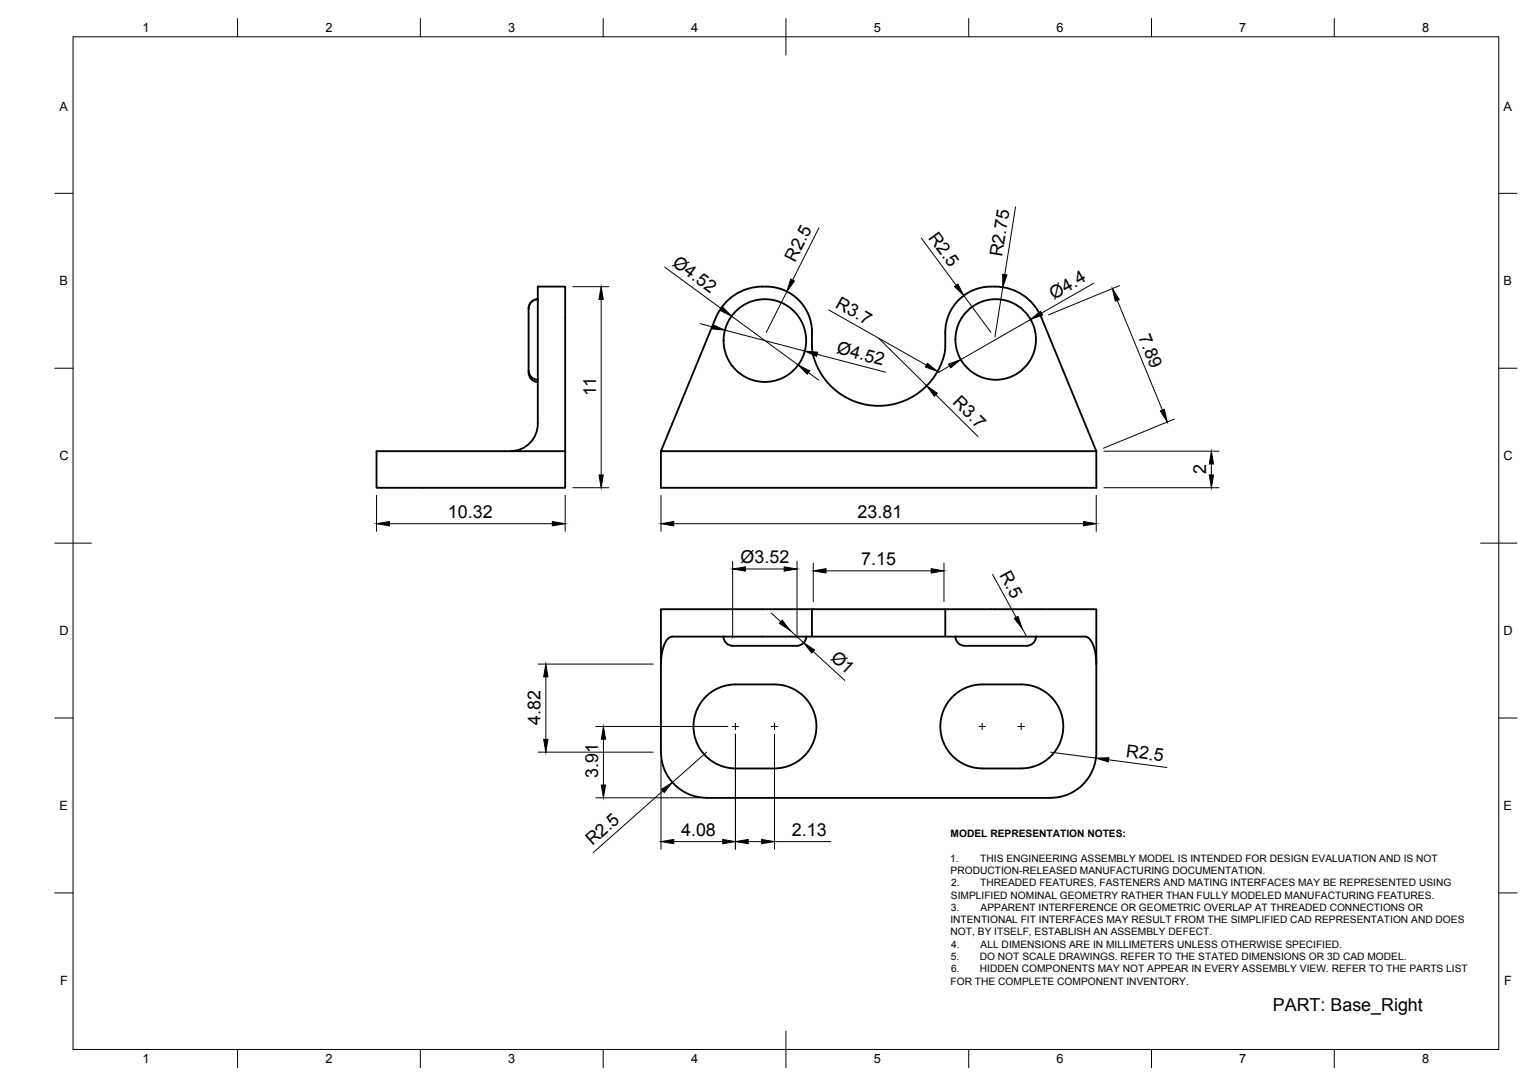
ISO-10303-21;
HEADER;
/* Generated by software containing ST-Developer
 * from STEP Tools, Inc. (www.steptools.com) 
 */

FILE_DESCRIPTION(
/* description */ (''),
/* implementation_level */ '2;1');

FILE_NAME(
/* name */ 'Base_Right.step',
/* time_stamp */ '2026-10-05T16:20:14-07:00',
/* author */ (''),
/* organization */ (''),
/* preprocessor_version */ 'ST-DEVELOPER v20.2',
/* originating_system */ 'Autodesk Translation Framework v15.15.0.0',
/* authorisation */ '');

FILE_SCHEMA (('AUTOMOTIVE_DESIGN { 1 0 10303 214 3 1 1 }'));
ENDSEC;

DATA;
#10=MECHANICAL_DESIGN_GEOMETRIC_PRESENTATION_REPRESENTATION('',(#249),#23577);
#209=ELLIPSE('',#4366,1.6218841056004,1.5);
#210=ELLIPSE('',#4367,1.6218841056004,1.5);
#215=TOROIDAL_SURFACE('',#4355,1.70133516896762,0.5);
#216=TOROIDAL_SURFACE('',#4360,1.75974879114541,0.5);
#231=SHAPE_REPRESENTATION_RELATIONSHIP('SRR','None',#23614,#240);
#240=ADVANCED_BREP_SHAPE_REPRESENTATION('',(#258),#23570);
#249=STYLED_ITEM('',(#23666),#258);
#258=MANIFOLD_SOLID_BREP('Body1',#4159);
#275=FACE_BOUND('',#681,.T.);
#276=FACE_BOUND('',#682,.T.);
#277=FACE_BOUND('',#686,.T.);
#278=FACE_BOUND('',#687,.T.);
#279=FACE_BOUND('',#714,.T.);
#280=FACE_BOUND('',#715,.T.);
#323=PLANE('',#4359);
#324=PLANE('',#4364);
#325=PLANE('',#4368);
#326=PLANE('',#4378);
#327=PLANE('',#4379);
#328=PLANE('',#4388);
#329=PLANE('',#4391);
#330=PLANE('',#4394);
#331=PLANE('',#4397);
#332=PLANE('',#4402);
#333=PLANE('',#4403);
#334=PLANE('',#4404);
#335=PLANE('',#4405);
#336=PLANE('',#4408);
#337=PLANE('',#4411);
#338=PLANE('',#4414);
#339=PLANE('',#4417);
#340=PLANE('',#4420);
#341=PLANE('',#4423);
#439=FACE_OUTER_BOUND('',#675,.T.);
#440=FACE_OUTER_BOUND('',#676,.T.);
#441=FACE_OUTER_BOUND('',#677,.T.);
#442=FACE_OUTER_BOUND('',#678,.T.);
#443=FACE_OUTER_BOUND('',#679,.T.);
#444=FACE_OUTER_BOUND('',#680,.T.);
#445=FACE_OUTER_BOUND('',#683,.T.);
#446=FACE_OUTER_BOUND('',#684,.T.);
#447=FACE_OUTER_BOUND('',#685,.T.);
#448=FACE_OUTER_BOUND('',#688,.T.);
#449=FACE_OUTER_BOUND('',#689,.T.);
#450=FACE_OUTER_BOUND('',#690,.T.);
#451=FACE_OUTER_BOUND('',#691,.T.);
#452=FACE_OUTER_BOUND('',#692,.T.);
#453=FACE_OUTER_BOUND('',#693,.T.);
#454=FACE_OUTER_BOUND('',#694,.T.);
#455=FACE_OUTER_BOUND('',#695,.T.);
#456=FACE_OUTER_BOUND('',#696,.T.);
#457=FACE_OUTER_BOUND('',#697,.T.);
#458=FACE_OUTER_BOUND('',#698,.T.);
#459=FACE_OUTER_BOUND('',#699,.T.);
#460=FACE_OUTER_BOUND('',#700,.T.);
#461=FACE_OUTER_BOUND('',#701,.T.);
#462=FACE_OUTER_BOUND('',#702,.T.);
#463=FACE_OUTER_BOUND('',#703,.T.);
#464=FACE_OUTER_BOUND('',#704,.T.);
#465=FACE_OUTER_BOUND('',#705,.T.);
#466=FACE_OUTER_BOUND('',#706,.T.);
#467=FACE_OUTER_BOUND('',#707,.T.);
#468=FACE_OUTER_BOUND('',#708,.T.);
#469=FACE_OUTER_BOUND('',#709,.T.);
#470=FACE_OUTER_BOUND('',#710,.T.);
#471=FACE_OUTER_BOUND('',#711,.T.);
#472=FACE_OUTER_BOUND('',#712,.T.);
#473=FACE_OUTER_BOUND('',#713,.T.);
#675=EDGE_LOOP('',(#2855,#2856,#2857,#2858));
#676=EDGE_LOOP('',(#2859));
#677=EDGE_LOOP('',(#2860,#2861,#2862,#2863));
#678=EDGE_LOOP('',(#2864));
#679=EDGE_LOOP('',(#2865,#2866,#2867,#2868));
#680=EDGE_LOOP('',(#2869,#2870,#2871,#2872,#2873,#2874));
#681=EDGE_LOOP('',(#2875,#2876,#2877,#2878));
#682=EDGE_LOOP('',(#2879,#2880,#2881,#2882));
#683=EDGE_LOOP('',(#2883,#2884,#2885,#2886));
#684=EDGE_LOOP('',(#2887,#2888,#2889,#2890));
#685=EDGE_LOOP('',(#2891,#2892,#2893,#2894,#2895,#2896,#2897,#2898,#2899,
#2900,#2901,#2902,#2903,#2904));
#686=EDGE_LOOP('',(#2905));
#687=EDGE_LOOP('',(#2906));
#688=EDGE_LOOP('',(#2907,#2908,#2909,#2910));
#689=EDGE_LOOP('',(#2911,#2912,#2913,#2914));
#690=EDGE_LOOP('',(#2915,#2916,#2917,#2918));
#691=EDGE_LOOP('',(#2919,#2920,#2921,#2922,#2923));
#692=EDGE_LOOP('',(#2924,#2925,#2926,#2927));
#693=EDGE_LOOP('',(#2928,#2929,#2930,#2931,#2932));
#694=EDGE_LOOP('',(#2933,#2934,#2935,#2936));
#695=EDGE_LOOP('',(#2937,#2938,#2939,#2940));
#696=EDGE_LOOP('',(#2941,#2942,#2943,#2944));
#697=EDGE_LOOP('',(#2945,#2946,#2947,#2948));
#698=EDGE_LOOP('',(#2949,#2950,#2951,#2952,#2953));
#699=EDGE_LOOP('',(#2954,#2955,#2956,#2957,#2958,#2959,#2960,#2961,#2962,
#2963,#2964,#2965,#2966,#2967,#2968,#2969));
#700=EDGE_LOOP('',(#2970,#2971,#2972,#2973));
#701=EDGE_LOOP('',(#2974,#2975,#2976,#2977));
#702=EDGE_LOOP('',(#2978,#2979,#2980,#2981));
#703=EDGE_LOOP('',(#2982,#2983,#2984,#2985));
#704=EDGE_LOOP('',(#2986,#2987,#2988,#2989));
#705=EDGE_LOOP('',(#2990,#2991,#2992,#2993));
#706=EDGE_LOOP('',(#2994,#2995,#2996,#2997));
#707=EDGE_LOOP('',(#2998,#2999,#3000,#3001));
#708=EDGE_LOOP('',(#3002,#3003,#3004,#3005));
#709=EDGE_LOOP('',(#3006,#3007,#3008,#3009,#3010));
#710=EDGE_LOOP('',(#3011,#3012,#3013,#3014));
#711=EDGE_LOOP('',(#3015,#3016,#3017,#3018));
#712=EDGE_LOOP('',(#3019,#3020,#3021,#3022));
#713=EDGE_LOOP('',(#3023,#3024,#3025,#3026,#3027,#3028));
#714=EDGE_LOOP('',(#3029,#3030,#3031,#3032));
#715=EDGE_LOOP('',(#3033,#3034,#3035,#3036));
#950=LINE('',#6022,#1235);
#951=LINE('',#6025,#1236);
#952=LINE('',#6028,#1237);
#953=LINE('',#6032,#1238);
#954=LINE('',#6035,#1239);
#955=LINE('',#6040,#1240);
#956=LINE('',#6043,#1241);
#957=LINE('',#6048,#1242);
#958=LINE('',#6051,#1243);
#959=LINE('',#6057,#1244);
#960=LINE('',#6060,#1245);
#961=LINE('',#6063,#1246);
#962=LINE('',#6065,#1247);
#963=LINE('',#6066,#1248);
#964=LINE('',#6069,#1249);
#965=LINE('',#6073,#1250);
#966=LINE('',#6077,#1251);
#967=LINE('',#6084,#1252);
#968=LINE('',#6087,#1253);
#969=LINE('',#6092,#1254);
#970=LINE('',#6093,#1255);
#971=LINE('',#6096,#1256);
#972=LINE('',#6097,#1257);
#973=LINE('',#6101,#1258);
#974=LINE('',#6104,#1259);
#975=LINE('',#6105,#1260);
#976=LINE('',#6108,#1261);
#977=LINE('',#6111,#1262);
#978=LINE('',#6114,#1263);
#979=LINE('',#6115,#1264);
#980=LINE('',#6120,#1265);
#981=LINE('',#6121,#1266);
#982=LINE('',#6123,#1267);
#983=LINE('',#6127,#1268);
#984=LINE('',#6132,#1269);
#985=LINE('',#6134,#1270);
#986=LINE('',#6135,#1271);
#987=LINE('',#6137,#1272);
#988=LINE('',#6139,#1273);
#989=LINE('',#6140,#1274);
#990=LINE('',#6145,#1275);
#991=LINE('',#6146,#1276);
#992=LINE('',#6147,#1277);
#993=LINE('',#6151,#1278);
#994=LINE('',#6154,#1279);
#995=LINE('',#6155,#1280);
#996=LINE('',#6161,#1281);
#997=LINE('',#6162,#1282);
#998=LINE('',#6163,#1283);
#999=LINE('',#6167,#1284);
#1000=LINE('',#6170,#1285);
#1001=LINE('',#6171,#1286);
#1002=LINE('',#6176,#1287);
#1003=LINE('',#6177,#1288);
#1004=LINE('',#6181,#1289);
#1005=LINE('',#6184,#1290);
#1006=LINE('',#6185,#1291);
#1235=VECTOR('',#4943,10.);
#1236=VECTOR('',#4946,10.);
#1237=VECTOR('',#4949,10.);
#1238=VECTOR('',#4952,10.);
#1239=VECTOR('',#4955,10.);
#1240=VECTOR('',#4958,10.);
#1241=VECTOR('',#4961,10.);
#1242=VECTOR('',#4964,10.);
#1243=VECTOR('',#4967,10.);
#1244=VECTOR('',#4972,10.);
#1245=VECTOR('',#4975,10.);
#1246=VECTOR('',#4978,10.);
#1247=VECTOR('',#4979,10.);
#1248=VECTOR('',#4980,10.);
#1249=VECTOR('',#4983,9.99999999999999);
#1250=VECTOR('',#4986,10.);
#1251=VECTOR('',#4989,10.);
#1252=VECTOR('',#4996,10.);
#1253=VECTOR('',#4999,9.99999999999999);
#1254=VECTOR('',#5004,10.);
#1255=VECTOR('',#5005,10.);
#1256=VECTOR('',#5008,10.);
#1257=VECTOR('',#5009,10.);
#1258=VECTOR('',#5014,10.);
#1259=VECTOR('',#5017,9.99999999999999);
#1260=VECTOR('',#5018,10.);
#1261=VECTOR('',#5021,10.);
#1262=VECTOR('',#5024,10.);
#1263=VECTOR('',#5027,10.);
#1264=VECTOR('',#5028,9.99999999999999);
#1265=VECTOR('',#5033,10.);
#1266=VECTOR('',#5034,10.);
#1267=VECTOR('',#5037,10.);
#1268=VECTOR('',#5042,10.);
#1269=VECTOR('',#5049,10.);
#1270=VECTOR('',#5050,10.);
#1271=VECTOR('',#5051,10.);
#1272=VECTOR('',#5054,10.);
#1273=VECTOR('',#5055,10.);
#1274=VECTOR('',#5056,10.);
#1275=VECTOR('',#5061,10.);
#1276=VECTOR('',#5062,10.);
#1277=VECTOR('',#5063,10.);
#1278=VECTOR('',#5068,10.);
#1279=VECTOR('',#5071,10.);
#1280=VECTOR('',#5072,10.);
#1281=VECTOR('',#5079,10.);
#1282=VECTOR('',#5080,10.);
#1283=VECTOR('',#5081,10.);
#1284=VECTOR('',#5086,10.);
#1285=VECTOR('',#5089,10.);
#1286=VECTOR('',#5090,10.);
#1287=VECTOR('',#5097,10.);
#1288=VECTOR('',#5098,10.);
#1289=VECTOR('',#5103,10.);
#1290=VECTOR('',#5106,10.);
#1291=VECTOR('',#5107,10.);
#1493=CIRCLE('',#4356,1.70133516896762);
#1494=CIRCLE('',#4357,0.5);
#1495=CIRCLE('',#4358,2.20133516896762);
#1496=CIRCLE('',#4361,1.75974879114541);
#1497=CIRCLE('',#4362,0.5);
#1498=CIRCLE('',#4363,2.25974879114541);
#1499=CIRCLE('',#4369,2.50000000000001);
#1500=CIRCLE('',#4370,2.5);
#1501=CIRCLE('',#4371,2.29663666580012);
#1502=CIRCLE('',#4372,2.29663666580012);
#1503=CIRCLE('',#4373,2.29663666580012);
#1504=CIRCLE('',#4374,2.29663666580012);
#1505=CIRCLE('',#4376,2.5);
#1506=CIRCLE('',#4377,2.5);
#1507=CIRCLE('',#4380,2.75);
#1508=CIRCLE('',#4381,2.5);
#1509=CIRCLE('',#4382,2.00000000000029);
#1510=CIRCLE('',#4383,3.70283120062258);
#1511=CIRCLE('',#4384,2.00000000000029);
#1512=CIRCLE('',#4385,2.75);
#1513=CIRCLE('',#4387,2.5);
#1514=CIRCLE('',#4390,2.75);
#1515=CIRCLE('',#4393,2.75);
#1516=CIRCLE('',#4396,2.00000000000029);
#1517=CIRCLE('',#4399,2.00000000000029);
#1518=CIRCLE('',#4401,3.70283120062258);
#1519=CIRCLE('',#4407,2.29663666580012);
#1520=CIRCLE('',#4410,2.29663666580012);
#1521=CIRCLE('',#4413,2.29663666580012);
#1522=CIRCLE('',#4416,2.29663666580012);
#1523=CIRCLE('',#4419,2.50000000000001);
#1524=CIRCLE('',#4422,2.5);
#1700=VERTEX_POINT('',#6004);
#1701=VERTEX_POINT('',#6006);
#1702=VERTEX_POINT('',#6011);
#1703=VERTEX_POINT('',#6013);
#1704=VERTEX_POINT('',#6018);
#1705=VERTEX_POINT('',#6019);
#1706=VERTEX_POINT('',#6021);
#1707=VERTEX_POINT('',#6023);
#1708=VERTEX_POINT('',#6027);
#1709=VERTEX_POINT('',#6029);
#1710=VERTEX_POINT('',#6031);
#1711=VERTEX_POINT('',#6033);
#1712=VERTEX_POINT('',#6036);
#1713=VERTEX_POINT('',#6037);
#1714=VERTEX_POINT('',#6039);
#1715=VERTEX_POINT('',#6041);
#1716=VERTEX_POINT('',#6044);
#1717=VERTEX_POINT('',#6045);
#1718=VERTEX_POINT('',#6047);
#1719=VERTEX_POINT('',#6049);
#1720=VERTEX_POINT('',#6053);
#1721=VERTEX_POINT('',#6054);
#1722=VERTEX_POINT('',#6056);
#1723=VERTEX_POINT('',#6058);
#1724=VERTEX_POINT('',#6062);
#1725=VERTEX_POINT('',#6064);
#1726=VERTEX_POINT('',#6068);
#1727=VERTEX_POINT('',#6070);
#1728=VERTEX_POINT('',#6072);
#1729=VERTEX_POINT('',#6074);
#1730=VERTEX_POINT('',#6076);
#1731=VERTEX_POINT('',#6078);
#1732=VERTEX_POINT('',#6080);
#1733=VERTEX_POINT('',#6082);
#1734=VERTEX_POINT('',#6085);
#1735=VERTEX_POINT('',#6089);
#1736=VERTEX_POINT('',#6090);
#1737=VERTEX_POINT('',#6095);
#1738=VERTEX_POINT('',#6099);
#1739=VERTEX_POINT('',#6103);
#1740=VERTEX_POINT('',#6107);
#1741=VERTEX_POINT('',#6109);
#1742=VERTEX_POINT('',#6113);
#1743=VERTEX_POINT('',#6117);
#1744=VERTEX_POINT('',#6118);
#1745=VERTEX_POINT('',#6125);
#1746=VERTEX_POINT('',#6131);
#1747=VERTEX_POINT('',#6133);
#1748=VERTEX_POINT('',#6138);
#1749=VERTEX_POINT('',#6143);
#1750=VERTEX_POINT('',#6144);
#1751=VERTEX_POINT('',#6149);
#1752=VERTEX_POINT('',#6153);
#1753=VERTEX_POINT('',#6159);
#1754=VERTEX_POINT('',#6160);
#1755=VERTEX_POINT('',#6165);
#1756=VERTEX_POINT('',#6169);
#1757=VERTEX_POINT('',#6175);
#1758=VERTEX_POINT('',#6179);
#1759=VERTEX_POINT('',#6183);
#2144=EDGE_CURVE('',#1700,#1700,#1493,.T.);
#2145=EDGE_CURVE('',#1700,#1701,#1494,.T.);
#2146=EDGE_CURVE('',#1701,#1701,#1495,.T.);
#2147=EDGE_CURVE('',#1702,#1702,#1496,.T.);
#2148=EDGE_CURVE('',#1702,#1703,#1497,.T.);
#2149=EDGE_CURVE('',#1703,#1703,#1498,.T.);
#2150=EDGE_CURVE('',#1704,#1705,#209,.T.);
#2151=EDGE_CURVE('',#1705,#1706,#950,.T.);
#2152=EDGE_CURVE('',#1707,#1706,#210,.F.);
#2153=EDGE_CURVE('',#1707,#1704,#951,.T.);
#2154=EDGE_CURVE('',#1708,#1707,#952,.T.);
#2155=EDGE_CURVE('',#1709,#1708,#1499,.T.);
#2156=EDGE_CURVE('',#1710,#1709,#953,.T.);
#2157=EDGE_CURVE('',#1711,#1710,#1500,.T.);
#2158=EDGE_CURVE('',#1704,#1711,#954,.T.);
#2159=EDGE_CURVE('',#1712,#1713,#1501,.T.);
#2160=EDGE_CURVE('',#1714,#1712,#955,.T.);
#2161=EDGE_CURVE('',#1715,#1714,#1502,.T.);
#2162=EDGE_CURVE('',#1713,#1715,#956,.T.);
#2163=EDGE_CURVE('',#1716,#1717,#1503,.T.);
#2164=EDGE_CURVE('',#1718,#1716,#957,.T.);
#2165=EDGE_CURVE('',#1719,#1718,#1504,.T.);
#2166=EDGE_CURVE('',#1717,#1719,#958,.T.);
#2167=EDGE_CURVE('',#1720,#1721,#1505,.T.);
#2168=EDGE_CURVE('',#1722,#1720,#959,.T.);
#2169=EDGE_CURVE('',#1723,#1722,#1506,.T.);
#2170=EDGE_CURVE('',#1721,#1723,#960,.T.);
#2171=EDGE_CURVE('',#1724,#1723,#961,.T.);
#2172=EDGE_CURVE('',#1724,#1725,#962,.T.);
#2173=EDGE_CURVE('',#1721,#1725,#963,.T.);
#2174=EDGE_CURVE('',#1726,#1705,#964,.T.);
#2175=EDGE_CURVE('',#1726,#1727,#1507,.T.);
#2176=EDGE_CURVE('',#1727,#1728,#965,.T.);
#2177=EDGE_CURVE('',#1728,#1729,#1508,.T.);
#2178=EDGE_CURVE('',#1730,#1729,#966,.T.);
#2179=EDGE_CURVE('',#1731,#1730,#1509,.T.);
#2180=EDGE_CURVE('',#1732,#1731,#1510,.T.);
#2181=EDGE_CURVE('',#1733,#1732,#1511,.T.);
#2182=EDGE_CURVE('',#1720,#1733,#967,.T.);
#2183=EDGE_CURVE('',#1725,#1734,#1512,.T.);
#2184=EDGE_CURVE('',#1706,#1734,#968,.T.);
#2185=EDGE_CURVE('',#1735,#1736,#1513,.T.);
#2186=EDGE_CURVE('',#1729,#1735,#969,.T.);
#2187=EDGE_CURVE('',#1736,#1728,#970,.T.);
#2188=EDGE_CURVE('',#1735,#1737,#971,.T.);
#2189=EDGE_CURVE('',#1730,#1737,#972,.T.);
#2190=EDGE_CURVE('',#1738,#1724,#1514,.T.);
#2191=EDGE_CURVE('',#1734,#1738,#973,.T.);
#2192=EDGE_CURVE('',#1738,#1739,#974,.T.);
#2193=EDGE_CURVE('',#1707,#1739,#975,.T.);
#2194=EDGE_CURVE('',#1740,#1726,#976,.T.);
#2195=EDGE_CURVE('',#1741,#1740,#1515,.T.);
#2196=EDGE_CURVE('',#1727,#1741,#977,.T.);
#2197=EDGE_CURVE('',#1704,#1742,#978,.T.);
#2198=EDGE_CURVE('',#1742,#1740,#979,.T.);
#2199=EDGE_CURVE('',#1743,#1744,#1516,.T.);
#2200=EDGE_CURVE('',#1733,#1744,#980,.T.);
#2201=EDGE_CURVE('',#1732,#1743,#981,.T.);
#2202=EDGE_CURVE('',#1744,#1722,#982,.T.);
#2203=EDGE_CURVE('',#1737,#1745,#1517,.T.);
#2204=EDGE_CURVE('',#1731,#1745,#983,.T.);
#2205=EDGE_CURVE('',#1745,#1743,#1518,.T.);
#2206=EDGE_CURVE('',#1746,#1739,#984,.T.);
#2207=EDGE_CURVE('',#1746,#1747,#985,.T.);
#2208=EDGE_CURVE('',#1747,#1708,#986,.T.);
#2209=EDGE_CURVE('',#1736,#1741,#987,.T.);
#2210=EDGE_CURVE('',#1748,#1742,#988,.T.);
#2211=EDGE_CURVE('',#1746,#1748,#989,.T.);
#2212=EDGE_CURVE('',#1749,#1750,#990,.T.);
#2213=EDGE_CURVE('',#1749,#1714,#991,.T.);
#2214=EDGE_CURVE('',#1750,#1712,#992,.T.);
#2215=EDGE_CURVE('',#1751,#1749,#1519,.T.);
#2216=EDGE_CURVE('',#1751,#1715,#993,.T.);
#2217=EDGE_CURVE('',#1752,#1751,#994,.T.);
#2218=EDGE_CURVE('',#1752,#1713,#995,.T.);
#2219=EDGE_CURVE('',#1750,#1752,#1520,.T.);
#2220=EDGE_CURVE('',#1753,#1754,#996,.T.);
#2221=EDGE_CURVE('',#1753,#1718,#997,.T.);
#2222=EDGE_CURVE('',#1754,#1716,#998,.T.);
#2223=EDGE_CURVE('',#1755,#1753,#1521,.T.);
#2224=EDGE_CURVE('',#1755,#1719,#999,.T.);
#2225=EDGE_CURVE('',#1756,#1755,#1000,.T.);
#2226=EDGE_CURVE('',#1756,#1717,#1001,.T.);
#2227=EDGE_CURVE('',#1754,#1756,#1522,.T.);
#2228=EDGE_CURVE('',#1757,#1711,#1002,.T.);
#2229=EDGE_CURVE('',#1748,#1757,#1003,.T.);
#2230=EDGE_CURVE('',#1758,#1747,#1523,.T.);
#2231=EDGE_CURVE('',#1758,#1709,#1004,.T.);
#2232=EDGE_CURVE('',#1758,#1759,#1005,.T.);
#2233=EDGE_CURVE('',#1759,#1710,#1006,.T.);
#2234=EDGE_CURVE('',#1757,#1759,#1524,.T.);
#2855=ORIENTED_EDGE('',*,*,#2144,.F.);
#2856=ORIENTED_EDGE('',*,*,#2145,.T.);
#2857=ORIENTED_EDGE('',*,*,#2146,.F.);
#2858=ORIENTED_EDGE('',*,*,#2145,.F.);
#2859=ORIENTED_EDGE('',*,*,#2144,.T.);
#2860=ORIENTED_EDGE('',*,*,#2147,.F.);
#2861=ORIENTED_EDGE('',*,*,#2148,.T.);
#2862=ORIENTED_EDGE('',*,*,#2149,.F.);
#2863=ORIENTED_EDGE('',*,*,#2148,.F.);
#2864=ORIENTED_EDGE('',*,*,#2147,.T.);
#2865=ORIENTED_EDGE('',*,*,#2150,.T.);
#2866=ORIENTED_EDGE('',*,*,#2151,.T.);
#2867=ORIENTED_EDGE('',*,*,#2152,.F.);
#2868=ORIENTED_EDGE('',*,*,#2153,.T.);
#2869=ORIENTED_EDGE('',*,*,#2153,.F.);
#2870=ORIENTED_EDGE('',*,*,#2154,.F.);
#2871=ORIENTED_EDGE('',*,*,#2155,.F.);
#2872=ORIENTED_EDGE('',*,*,#2156,.F.);
#2873=ORIENTED_EDGE('',*,*,#2157,.F.);
#2874=ORIENTED_EDGE('',*,*,#2158,.F.);
#2875=ORIENTED_EDGE('',*,*,#2159,.F.);
#2876=ORIENTED_EDGE('',*,*,#2160,.F.);
#2877=ORIENTED_EDGE('',*,*,#2161,.F.);
#2878=ORIENTED_EDGE('',*,*,#2162,.F.);
#2879=ORIENTED_EDGE('',*,*,#2163,.F.);
#2880=ORIENTED_EDGE('',*,*,#2164,.F.);
#2881=ORIENTED_EDGE('',*,*,#2165,.F.);
#2882=ORIENTED_EDGE('',*,*,#2166,.F.);
#2883=ORIENTED_EDGE('',*,*,#2167,.F.);
#2884=ORIENTED_EDGE('',*,*,#2168,.F.);
#2885=ORIENTED_EDGE('',*,*,#2169,.F.);
#2886=ORIENTED_EDGE('',*,*,#2170,.F.);
#2887=ORIENTED_EDGE('',*,*,#2170,.T.);
#2888=ORIENTED_EDGE('',*,*,#2171,.F.);
#2889=ORIENTED_EDGE('',*,*,#2172,.T.);
#2890=ORIENTED_EDGE('',*,*,#2173,.F.);
#2891=ORIENTED_EDGE('',*,*,#2151,.F.);
#2892=ORIENTED_EDGE('',*,*,#2174,.F.);
#2893=ORIENTED_EDGE('',*,*,#2175,.T.);
#2894=ORIENTED_EDGE('',*,*,#2176,.T.);
#2895=ORIENTED_EDGE('',*,*,#2177,.T.);
#2896=ORIENTED_EDGE('',*,*,#2178,.F.);
#2897=ORIENTED_EDGE('',*,*,#2179,.F.);
#2898=ORIENTED_EDGE('',*,*,#2180,.F.);
#2899=ORIENTED_EDGE('',*,*,#2181,.F.);
#2900=ORIENTED_EDGE('',*,*,#2182,.F.);
#2901=ORIENTED_EDGE('',*,*,#2167,.T.);
#2902=ORIENTED_EDGE('',*,*,#2173,.T.);
#2903=ORIENTED_EDGE('',*,*,#2183,.T.);
#2904=ORIENTED_EDGE('',*,*,#2184,.F.);
#2905=ORIENTED_EDGE('',*,*,#2146,.T.);
#2906=ORIENTED_EDGE('',*,*,#2149,.T.);
#2907=ORIENTED_EDGE('',*,*,#2185,.F.);
#2908=ORIENTED_EDGE('',*,*,#2186,.F.);
#2909=ORIENTED_EDGE('',*,*,#2177,.F.);
#2910=ORIENTED_EDGE('',*,*,#2187,.F.);
#2911=ORIENTED_EDGE('',*,*,#2186,.T.);
#2912=ORIENTED_EDGE('',*,*,#2188,.T.);
#2913=ORIENTED_EDGE('',*,*,#2189,.F.);
#2914=ORIENTED_EDGE('',*,*,#2178,.T.);
#2915=ORIENTED_EDGE('',*,*,#2190,.F.);
#2916=ORIENTED_EDGE('',*,*,#2191,.F.);
#2917=ORIENTED_EDGE('',*,*,#2183,.F.);
#2918=ORIENTED_EDGE('',*,*,#2172,.F.);
#2919=ORIENTED_EDGE('',*,*,#2191,.T.);
#2920=ORIENTED_EDGE('',*,*,#2192,.T.);
#2921=ORIENTED_EDGE('',*,*,#2193,.F.);
#2922=ORIENTED_EDGE('',*,*,#2152,.T.);
#2923=ORIENTED_EDGE('',*,*,#2184,.T.);
#2924=ORIENTED_EDGE('',*,*,#2175,.F.);
#2925=ORIENTED_EDGE('',*,*,#2194,.F.);
#2926=ORIENTED_EDGE('',*,*,#2195,.F.);
#2927=ORIENTED_EDGE('',*,*,#2196,.F.);
#2928=ORIENTED_EDGE('',*,*,#2194,.T.);
#2929=ORIENTED_EDGE('',*,*,#2174,.T.);
#2930=ORIENTED_EDGE('',*,*,#2150,.F.);
#2931=ORIENTED_EDGE('',*,*,#2197,.T.);
#2932=ORIENTED_EDGE('',*,*,#2198,.T.);
#2933=ORIENTED_EDGE('',*,*,#2199,.T.);
#2934=ORIENTED_EDGE('',*,*,#2200,.F.);
#2935=ORIENTED_EDGE('',*,*,#2181,.T.);
#2936=ORIENTED_EDGE('',*,*,#2201,.T.);
#2937=ORIENTED_EDGE('',*,*,#2168,.T.);
#2938=ORIENTED_EDGE('',*,*,#2182,.T.);
#2939=ORIENTED_EDGE('',*,*,#2200,.T.);
#2940=ORIENTED_EDGE('',*,*,#2202,.T.);
#2941=ORIENTED_EDGE('',*,*,#2203,.T.);
#2942=ORIENTED_EDGE('',*,*,#2204,.F.);
#2943=ORIENTED_EDGE('',*,*,#2179,.T.);
#2944=ORIENTED_EDGE('',*,*,#2189,.T.);
#2945=ORIENTED_EDGE('',*,*,#2205,.T.);
#2946=ORIENTED_EDGE('',*,*,#2201,.F.);
#2947=ORIENTED_EDGE('',*,*,#2180,.T.);
#2948=ORIENTED_EDGE('',*,*,#2204,.T.);
#2949=ORIENTED_EDGE('',*,*,#2193,.T.);
#2950=ORIENTED_EDGE('',*,*,#2206,.F.);
#2951=ORIENTED_EDGE('',*,*,#2207,.T.);
#2952=ORIENTED_EDGE('',*,*,#2208,.T.);
#2953=ORIENTED_EDGE('',*,*,#2154,.T.);
#2954=ORIENTED_EDGE('',*,*,#2169,.T.);
#2955=ORIENTED_EDGE('',*,*,#2202,.F.);
#2956=ORIENTED_EDGE('',*,*,#2199,.F.);
#2957=ORIENTED_EDGE('',*,*,#2205,.F.);
#2958=ORIENTED_EDGE('',*,*,#2203,.F.);
#2959=ORIENTED_EDGE('',*,*,#2188,.F.);
#2960=ORIENTED_EDGE('',*,*,#2185,.T.);
#2961=ORIENTED_EDGE('',*,*,#2209,.T.);
#2962=ORIENTED_EDGE('',*,*,#2195,.T.);
#2963=ORIENTED_EDGE('',*,*,#2198,.F.);
#2964=ORIENTED_EDGE('',*,*,#2210,.F.);
#2965=ORIENTED_EDGE('',*,*,#2211,.F.);
#2966=ORIENTED_EDGE('',*,*,#2206,.T.);
#2967=ORIENTED_EDGE('',*,*,#2192,.F.);
#2968=ORIENTED_EDGE('',*,*,#2190,.T.);
#2969=ORIENTED_EDGE('',*,*,#2171,.T.);
#2970=ORIENTED_EDGE('',*,*,#2187,.T.);
#2971=ORIENTED_EDGE('',*,*,#2176,.F.);
#2972=ORIENTED_EDGE('',*,*,#2196,.T.);
#2973=ORIENTED_EDGE('',*,*,#2209,.F.);
#2974=ORIENTED_EDGE('',*,*,#2212,.F.);
#2975=ORIENTED_EDGE('',*,*,#2213,.T.);
#2976=ORIENTED_EDGE('',*,*,#2160,.T.);
#2977=ORIENTED_EDGE('',*,*,#2214,.F.);
#2978=ORIENTED_EDGE('',*,*,#2215,.F.);
#2979=ORIENTED_EDGE('',*,*,#2216,.T.);
#2980=ORIENTED_EDGE('',*,*,#2161,.T.);
#2981=ORIENTED_EDGE('',*,*,#2213,.F.);
#2982=ORIENTED_EDGE('',*,*,#2217,.F.);
#2983=ORIENTED_EDGE('',*,*,#2218,.T.);
#2984=ORIENTED_EDGE('',*,*,#2162,.T.);
#2985=ORIENTED_EDGE('',*,*,#2216,.F.);
#2986=ORIENTED_EDGE('',*,*,#2219,.F.);
#2987=ORIENTED_EDGE('',*,*,#2214,.T.);
#2988=ORIENTED_EDGE('',*,*,#2159,.T.);
#2989=ORIENTED_EDGE('',*,*,#2218,.F.);
#2990=ORIENTED_EDGE('',*,*,#2220,.F.);
#2991=ORIENTED_EDGE('',*,*,#2221,.T.);
#2992=ORIENTED_EDGE('',*,*,#2164,.T.);
#2993=ORIENTED_EDGE('',*,*,#2222,.F.);
#2994=ORIENTED_EDGE('',*,*,#2223,.F.);
#2995=ORIENTED_EDGE('',*,*,#2224,.T.);
#2996=ORIENTED_EDGE('',*,*,#2165,.T.);
#2997=ORIENTED_EDGE('',*,*,#2221,.F.);
#2998=ORIENTED_EDGE('',*,*,#2225,.F.);
#2999=ORIENTED_EDGE('',*,*,#2226,.T.);
#3000=ORIENTED_EDGE('',*,*,#2166,.T.);
#3001=ORIENTED_EDGE('',*,*,#2224,.F.);
#3002=ORIENTED_EDGE('',*,*,#2227,.F.);
#3003=ORIENTED_EDGE('',*,*,#2222,.T.);
#3004=ORIENTED_EDGE('',*,*,#2163,.T.);
#3005=ORIENTED_EDGE('',*,*,#2226,.F.);
#3006=ORIENTED_EDGE('',*,*,#2197,.F.);
#3007=ORIENTED_EDGE('',*,*,#2158,.T.);
#3008=ORIENTED_EDGE('',*,*,#2228,.F.);
#3009=ORIENTED_EDGE('',*,*,#2229,.F.);
#3010=ORIENTED_EDGE('',*,*,#2210,.T.);
#3011=ORIENTED_EDGE('',*,*,#2230,.F.);
#3012=ORIENTED_EDGE('',*,*,#2231,.T.);
#3013=ORIENTED_EDGE('',*,*,#2155,.T.);
#3014=ORIENTED_EDGE('',*,*,#2208,.F.);
#3015=ORIENTED_EDGE('',*,*,#2232,.T.);
#3016=ORIENTED_EDGE('',*,*,#2233,.T.);
#3017=ORIENTED_EDGE('',*,*,#2156,.T.);
#3018=ORIENTED_EDGE('',*,*,#2231,.F.);
#3019=ORIENTED_EDGE('',*,*,#2234,.F.);
#3020=ORIENTED_EDGE('',*,*,#2228,.T.);
#3021=ORIENTED_EDGE('',*,*,#2157,.T.);
#3022=ORIENTED_EDGE('',*,*,#2233,.F.);
#3023=ORIENTED_EDGE('',*,*,#2234,.T.);
#3024=ORIENTED_EDGE('',*,*,#2232,.F.);
#3025=ORIENTED_EDGE('',*,*,#2230,.T.);
#3026=ORIENTED_EDGE('',*,*,#2207,.F.);
#3027=ORIENTED_EDGE('',*,*,#2211,.T.);
#3028=ORIENTED_EDGE('',*,*,#2229,.T.);
#3029=ORIENTED_EDGE('',*,*,#2227,.T.);
#3030=ORIENTED_EDGE('',*,*,#2225,.T.);
#3031=ORIENTED_EDGE('',*,*,#2223,.T.);
#3032=ORIENTED_EDGE('',*,*,#2220,.T.);
#3033=ORIENTED_EDGE('',*,*,#2219,.T.);
#3034=ORIENTED_EDGE('',*,*,#2217,.T.);
#3035=ORIENTED_EDGE('',*,*,#2215,.T.);
#3036=ORIENTED_EDGE('',*,*,#2212,.T.);
#3859=CYLINDRICAL_SURFACE('',#4365,1.5);
#3860=CYLINDRICAL_SURFACE('',#4375,2.5);
#3861=CYLINDRICAL_SURFACE('',#4386,2.5);
#3862=CYLINDRICAL_SURFACE('',#4389,2.75);
#3863=CYLINDRICAL_SURFACE('',#4392,2.75);
#3864=CYLINDRICAL_SURFACE('',#4395,2.00000000000029);
#3865=CYLINDRICAL_SURFACE('',#4398,2.00000000000029);
#3866=CYLINDRICAL_SURFACE('',#4400,3.70283120062258);
#3867=CYLINDRICAL_SURFACE('',#4406,2.29663666580012);
#3868=CYLINDRICAL_SURFACE('',#4409,2.29663666580012);
#3869=CYLINDRICAL_SURFACE('',#4412,2.29663666580012);
#3870=CYLINDRICAL_SURFACE('',#4415,2.29663666580012);
#3871=CYLINDRICAL_SURFACE('',#4418,2.50000000000001);
#3872=CYLINDRICAL_SURFACE('',#4421,2.5);
#3974=ADVANCED_FACE('',(#439),#215,.T.);
#3975=ADVANCED_FACE('',(#440),#323,.F.);
#3976=ADVANCED_FACE('',(#441),#216,.T.);
#3977=ADVANCED_FACE('',(#442),#324,.F.);
#3978=ADVANCED_FACE('',(#443),#3859,.F.);
#3979=ADVANCED_FACE('',(#444,#275,#276),#325,.F.);
#3980=ADVANCED_FACE('',(#445),#3860,.T.);
#3981=ADVANCED_FACE('',(#446),#326,.F.);
#3982=ADVANCED_FACE('',(#447,#277,#278),#327,.F.);
#3983=ADVANCED_FACE('',(#448),#3861,.T.);
#3984=ADVANCED_FACE('',(#449),#328,.T.);
#3985=ADVANCED_FACE('',(#450),#3862,.T.);
#3986=ADVANCED_FACE('',(#451),#329,.T.);
#3987=ADVANCED_FACE('',(#452),#3863,.T.);
#3988=ADVANCED_FACE('',(#453),#330,.T.);
#3989=ADVANCED_FACE('',(#454),#3864,.F.);
#3990=ADVANCED_FACE('',(#455),#331,.T.);
#3991=ADVANCED_FACE('',(#456),#3865,.F.);
#3992=ADVANCED_FACE('',(#457),#3866,.F.);
#3993=ADVANCED_FACE('',(#458),#332,.F.);
#3994=ADVANCED_FACE('',(#459),#333,.F.);
#3995=ADVANCED_FACE('',(#460),#334,.F.);
#3996=ADVANCED_FACE('',(#461),#335,.F.);
#3997=ADVANCED_FACE('',(#462),#3867,.F.);
#3998=ADVANCED_FACE('',(#463),#336,.F.);
#3999=ADVANCED_FACE('',(#464),#3868,.F.);
#4000=ADVANCED_FACE('',(#465),#337,.F.);
#4001=ADVANCED_FACE('',(#466),#3869,.F.);
#4002=ADVANCED_FACE('',(#467),#338,.F.);
#4003=ADVANCED_FACE('',(#468),#3870,.F.);
#4004=ADVANCED_FACE('',(#469),#339,.F.);
#4005=ADVANCED_FACE('',(#470),#3871,.T.);
#4006=ADVANCED_FACE('',(#471),#340,.F.);
#4007=ADVANCED_FACE('',(#472),#3872,.T.);
#4008=ADVANCED_FACE('',(#473,#279,#280),#341,.T.);
#4159=CLOSED_SHELL('',(#3974,#3975,#3976,#3977,#3978,#3979,#3980,#3981,
#3982,#3983,#3984,#3985,#3986,#3987,#3988,#3989,#3990,#3991,#3992,#3993,
#3994,#3995,#3996,#3997,#3998,#3999,#4000,#4001,#4002,#4003,#4004,#4005,
#4006,#4007,#4008));
#4354=AXIS2_PLACEMENT_3D('',#6002,#4917,#4918);
#4355=AXIS2_PLACEMENT_3D('',#6003,#4919,#4920);
#4356=AXIS2_PLACEMENT_3D('',#6005,#4921,#4922);
#4357=AXIS2_PLACEMENT_3D('',#6007,#4923,#4924);
#4358=AXIS2_PLACEMENT_3D('',#6008,#4925,#4926);
#4359=AXIS2_PLACEMENT_3D('',#6009,#4927,#4928);
#4360=AXIS2_PLACEMENT_3D('',#6010,#4929,#4930);
#4361=AXIS2_PLACEMENT_3D('',#6012,#4931,#4932);
#4362=AXIS2_PLACEMENT_3D('',#6014,#4933,#4934);
#4363=AXIS2_PLACEMENT_3D('',#6015,#4935,#4936);
#4364=AXIS2_PLACEMENT_3D('',#6016,#4937,#4938);
#4365=AXIS2_PLACEMENT_3D('',#6017,#4939,#4940);
#4366=AXIS2_PLACEMENT_3D('',#6020,#4941,#4942);
#4367=AXIS2_PLACEMENT_3D('',#6024,#4944,#4945);
#4368=AXIS2_PLACEMENT_3D('',#6026,#4947,#4948);
#4369=AXIS2_PLACEMENT_3D('',#6030,#4950,#4951);
#4370=AXIS2_PLACEMENT_3D('',#6034,#4953,#4954);
#4371=AXIS2_PLACEMENT_3D('',#6038,#4956,#4957);
#4372=AXIS2_PLACEMENT_3D('',#6042,#4959,#4960);
#4373=AXIS2_PLACEMENT_3D('',#6046,#4962,#4963);
#4374=AXIS2_PLACEMENT_3D('',#6050,#4965,#4966);
#4375=AXIS2_PLACEMENT_3D('',#6052,#4968,#4969);
#4376=AXIS2_PLACEMENT_3D('',#6055,#4970,#4971);
#4377=AXIS2_PLACEMENT_3D('',#6059,#4973,#4974);
#4378=AXIS2_PLACEMENT_3D('',#6061,#4976,#4977);
#4379=AXIS2_PLACEMENT_3D('',#6067,#4981,#4982);
#4380=AXIS2_PLACEMENT_3D('',#6071,#4984,#4985);
#4381=AXIS2_PLACEMENT_3D('',#6075,#4987,#4988);
#4382=AXIS2_PLACEMENT_3D('',#6079,#4990,#4991);
#4383=AXIS2_PLACEMENT_3D('',#6081,#4992,#4993);
#4384=AXIS2_PLACEMENT_3D('',#6083,#4994,#4995);
#4385=AXIS2_PLACEMENT_3D('',#6086,#4997,#4998);
#4386=AXIS2_PLACEMENT_3D('',#6088,#5000,#5001);
#4387=AXIS2_PLACEMENT_3D('',#6091,#5002,#5003);
#4388=AXIS2_PLACEMENT_3D('',#6094,#5006,#5007);
#4389=AXIS2_PLACEMENT_3D('',#6098,#5010,#5011);
#4390=AXIS2_PLACEMENT_3D('',#6100,#5012,#5013);
#4391=AXIS2_PLACEMENT_3D('',#6102,#5015,#5016);
#4392=AXIS2_PLACEMENT_3D('',#6106,#5019,#5020);
#4393=AXIS2_PLACEMENT_3D('',#6110,#5022,#5023);
#4394=AXIS2_PLACEMENT_3D('',#6112,#5025,#5026);
#4395=AXIS2_PLACEMENT_3D('',#6116,#5029,#5030);
#4396=AXIS2_PLACEMENT_3D('',#6119,#5031,#5032);
#4397=AXIS2_PLACEMENT_3D('',#6122,#5035,#5036);
#4398=AXIS2_PLACEMENT_3D('',#6124,#5038,#5039);
#4399=AXIS2_PLACEMENT_3D('',#6126,#5040,#5041);
#4400=AXIS2_PLACEMENT_3D('',#6128,#5043,#5044);
#4401=AXIS2_PLACEMENT_3D('',#6129,#5045,#5046);
#4402=AXIS2_PLACEMENT_3D('',#6130,#5047,#5048);
#4403=AXIS2_PLACEMENT_3D('',#6136,#5052,#5053);
#4404=AXIS2_PLACEMENT_3D('',#6141,#5057,#5058);
#4405=AXIS2_PLACEMENT_3D('',#6142,#5059,#5060);
#4406=AXIS2_PLACEMENT_3D('',#6148,#5064,#5065);
#4407=AXIS2_PLACEMENT_3D('',#6150,#5066,#5067);
#4408=AXIS2_PLACEMENT_3D('',#6152,#5069,#5070);
#4409=AXIS2_PLACEMENT_3D('',#6156,#5073,#5074);
#4410=AXIS2_PLACEMENT_3D('',#6157,#5075,#5076);
#4411=AXIS2_PLACEMENT_3D('',#6158,#5077,#5078);
#4412=AXIS2_PLACEMENT_3D('',#6164,#5082,#5083);
#4413=AXIS2_PLACEMENT_3D('',#6166,#5084,#5085);
#4414=AXIS2_PLACEMENT_3D('',#6168,#5087,#5088);
#4415=AXIS2_PLACEMENT_3D('',#6172,#5091,#5092);
#4416=AXIS2_PLACEMENT_3D('',#6173,#5093,#5094);
#4417=AXIS2_PLACEMENT_3D('',#6174,#5095,#5096);
#4418=AXIS2_PLACEMENT_3D('',#6178,#5099,#5100);
#4419=AXIS2_PLACEMENT_3D('',#6180,#5101,#5102);
#4420=AXIS2_PLACEMENT_3D('',#6182,#5104,#5105);
#4421=AXIS2_PLACEMENT_3D('',#6186,#5108,#5109);
#4422=AXIS2_PLACEMENT_3D('',#6187,#5110,#5111);
#4423=AXIS2_PLACEMENT_3D('',#6188,#5112,#5113);
#4917=DIRECTION('axis',(0.,0.,1.));
#4918=DIRECTION('refdir',(1.,0.,0.));
#4919=DIRECTION('center_axis',(0.,1.,0.));
#4920=DIRECTION('ref_axis',(0.,0.,-1.));
#4921=DIRECTION('center_axis',(0.,1.,0.));
#4922=DIRECTION('ref_axis',(1.,0.,0.));
#4923=DIRECTION('center_axis',(1.,0.,0.));
#4924=DIRECTION('ref_axis',(0.,0.,1.));
#4925=DIRECTION('center_axis',(0.,-1.,0.));
#4926=DIRECTION('ref_axis',(0.,0.,1.));
#4927=DIRECTION('center_axis',(0.,-1.,0.));
#4928=DIRECTION('ref_axis',(1.,0.,0.));
#4929=DIRECTION('center_axis',(0.,1.,0.));
#4930=DIRECTION('ref_axis',(0.,0.,-1.));
#4931=DIRECTION('center_axis',(0.,1.,0.));
#4932=DIRECTION('ref_axis',(1.,0.,0.));
#4933=DIRECTION('center_axis',(1.,0.,0.));
#4934=DIRECTION('ref_axis',(0.,0.,1.));
#4935=DIRECTION('center_axis',(0.,-1.,0.));
#4936=DIRECTION('ref_axis',(0.,0.,1.));
#4937=DIRECTION('center_axis',(0.,-1.,0.));
#4938=DIRECTION('ref_axis',(1.,0.,0.));
#4939=DIRECTION('center_axis',(-1.,0.,0.));
#4940=DIRECTION('ref_axis',(0.,-0.707106781186547,-0.707106781186548));
#4941=DIRECTION('center_axis',(-0.924850298995146,0.,0.380331335086382));
#4942=DIRECTION('ref_axis',(-0.380331335086382,3.4226336542529E-16,-0.924850298995146));
#4943=DIRECTION('',(1.,0.,0.));
#4944=DIRECTION('center_axis',(0.924850298995146,0.,0.380331335086382));
#4945=DIRECTION('ref_axis',(0.380331335086382,0.,-0.924850298995146));
#4946=DIRECTION('',(-1.,0.,0.));
#4947=DIRECTION('center_axis',(0.,0.,-1.));
#4948=DIRECTION('ref_axis',(1.,0.,0.));
#4949=DIRECTION('',(0.,-1.,0.));
#4950=DIRECTION('center_axis',(0.,0.,-1.));
#4951=DIRECTION('ref_axis',(3.55271367880049E-15,1.,0.));
#4952=DIRECTION('',(1.,2.36032074788338E-16,0.));
#4953=DIRECTION('center_axis',(0.,0.,-1.));
#4954=DIRECTION('ref_axis',(-1.,0.,0.));
#4955=DIRECTION('',(3.51417407375166E-16,1.,0.));
#4956=DIRECTION('center_axis',(0.,0.,1.));
#4957=DIRECTION('ref_axis',(0.,-1.,0.));
#4958=DIRECTION('',(-1.,0.,0.));
#4959=DIRECTION('center_axis',(0.,0.,1.));
#4960=DIRECTION('ref_axis',(0.,1.,0.));
#4961=DIRECTION('',(1.,0.,0.));
#4962=DIRECTION('center_axis',(0.,0.,1.));
#4963=DIRECTION('ref_axis',(0.,-1.,0.));
#4964=DIRECTION('',(-1.,0.,0.));
#4965=DIRECTION('center_axis',(0.,0.,1.));
#4966=DIRECTION('ref_axis',(0.,1.,0.));
#4967=DIRECTION('',(1.,0.,0.));
#4968=DIRECTION('center_axis',(0.,-1.,0.));
#4969=DIRECTION('ref_axis',(-0.707106781186548,0.,0.707106781186548));
#4970=DIRECTION('center_axis',(0.,1.,0.));
#4971=DIRECTION('ref_axis',(-0.707106781186548,0.,0.707106781186548));
#4972=DIRECTION('',(0.,1.,0.));
#4973=DIRECTION('center_axis',(0.,-1.,0.));
#4974=DIRECTION('ref_axis',(-0.707106781186548,0.,0.707106781186548));
#4975=DIRECTION('',(0.,-1.,0.));
#4976=DIRECTION('center_axis',(0.,0.,-1.));
#4977=DIRECTION('ref_axis',(1.,0.,0.));
#4978=DIRECTION('',(-1.,0.,0.));
#4979=DIRECTION('',(0.,1.,0.));
#4980=DIRECTION('',(1.,0.,0.));
#4981=DIRECTION('center_axis',(0.,-1.,0.));
#4982=DIRECTION('ref_axis',(1.,0.,0.));
#4983=DIRECTION('',(-0.380331335086382,0.,-0.924850298995146));
#4984=DIRECTION('center_axis',(0.,1.,0.));
#4985=DIRECTION('ref_axis',(-0.556627642555424,0.,0.830762100449455));
#4986=DIRECTION('',(1.,0.,0.));
#4987=DIRECTION('center_axis',(0.,1.,0.));
#4988=DIRECTION('ref_axis',(0.707106781186548,0.,0.707106781186548));
#4989=DIRECTION('',(0.,0.,1.));
#4990=DIRECTION('center_axis',(0.,1.,0.));
#4991=DIRECTION('ref_axis',(-1.,0.,-1.85962356624686E-14));
#4992=DIRECTION('center_axis',(0.,1.,0.));
#4993=DIRECTION('ref_axis',(-0.965748659616478,0.,-0.259479337229339));
#4994=DIRECTION('center_axis',(0.,1.,0.));
#4995=DIRECTION('ref_axis',(0.965748659616483,0.,-0.259479337229319));
#4996=DIRECTION('',(0.,0.,-1.));
#4997=DIRECTION('center_axis',(0.,1.,0.));
#4998=DIRECTION('ref_axis',(0.556627642555425,0.,0.830762100449455));
#4999=DIRECTION('',(-0.380331335086382,0.,0.924850298995146));
#5000=DIRECTION('center_axis',(0.,1.,0.));
#5001=DIRECTION('ref_axis',(0.707106781186548,0.,0.707106781186548));
#5002=DIRECTION('center_axis',(0.,-1.,0.));
#5003=DIRECTION('ref_axis',(0.707106781186548,0.,0.707106781186548));
#5004=DIRECTION('',(0.,-1.,0.));
#5005=DIRECTION('',(0.,1.,0.));
#5006=DIRECTION('center_axis',(1.,0.,0.));
#5007=DIRECTION('ref_axis',(0.,0.,1.));
#5008=DIRECTION('',(0.,0.,-1.));
#5009=DIRECTION('',(0.,-1.,0.));
#5010=DIRECTION('center_axis',(0.,1.,0.));
#5011=DIRECTION('ref_axis',(0.556627642555425,0.,0.830762100449455));
#5012=DIRECTION('center_axis',(0.,-1.,0.));
#5013=DIRECTION('ref_axis',(0.556627642555425,0.,0.830762100449455));
#5014=DIRECTION('',(0.,-1.,0.));
#5015=DIRECTION('center_axis',(0.924850298995146,0.,0.380331335086382));
#5016=DIRECTION('ref_axis',(-0.380331335086382,0.,0.924850298995145));
#5017=DIRECTION('',(0.380331335086382,0.,-0.924850298995146));
#5018=DIRECTION('',(0.,-1.,0.));
#5019=DIRECTION('center_axis',(0.,-1.,0.));
#5020=DIRECTION('ref_axis',(-0.556627642555424,0.,0.830762100449455));
#5021=DIRECTION('',(0.,1.,0.));
#5022=DIRECTION('center_axis',(0.,-1.,0.));
#5023=DIRECTION('ref_axis',(-0.556627642555424,0.,0.830762100449455));
#5024=DIRECTION('',(0.,-1.,0.));
#5025=DIRECTION('center_axis',(-0.924850298995146,0.,0.380331335086382));
#5026=DIRECTION('ref_axis',(-0.380331335086382,0.,-0.924850298995145));
#5027=DIRECTION('',(-3.51417407375166E-16,-1.,-8.54540408060787E-16));
#5028=DIRECTION('',(0.380331335086382,0.,0.924850298995146));
#5029=DIRECTION('center_axis',(0.,1.,0.));
#5030=DIRECTION('ref_axis',(0.965748659616483,0.,-0.259479337229319));
#5031=DIRECTION('center_axis',(0.,-1.,0.));
#5032=DIRECTION('ref_axis',(0.965748659616483,0.,-0.259479337229319));
#5033=DIRECTION('',(0.,-1.,0.));
#5034=DIRECTION('',(0.,-1.,0.));
#5035=DIRECTION('center_axis',(-1.,0.,0.));
#5036=DIRECTION('ref_axis',(0.,0.,-1.));
#5037=DIRECTION('',(0.,0.,1.));
#5038=DIRECTION('center_axis',(0.,1.,0.));
#5039=DIRECTION('ref_axis',(-1.,0.,-1.85962356624686E-14));
#5040=DIRECTION('center_axis',(0.,-1.,0.));
#5041=DIRECTION('ref_axis',(-1.,0.,-1.85962356624686E-14));
#5042=DIRECTION('',(0.,-1.,0.));
#5043=DIRECTION('center_axis',(0.,1.,0.));
#5044=DIRECTION('ref_axis',(-0.965748659616478,0.,-0.259479337229339));
#5045=DIRECTION('center_axis',(0.,-1.,0.));
#5046=DIRECTION('ref_axis',(-0.965748659616478,0.,-0.259479337229339));
#5047=DIRECTION('center_axis',(-1.,0.,0.));
#5048=DIRECTION('ref_axis',(0.,-1.,0.));
#5049=DIRECTION('',(0.,0.,1.));
#5050=DIRECTION('',(0.,1.,0.));
#5051=DIRECTION('',(0.,0.,1.));
#5052=DIRECTION('center_axis',(0.,1.,0.));
#5053=DIRECTION('ref_axis',(-1.,0.,0.));
#5054=DIRECTION('',(-1.,0.,0.));
#5055=DIRECTION('',(0.,0.,1.));
#5056=DIRECTION('',(-1.,0.,0.));
#5057=DIRECTION('center_axis',(0.,0.,-1.));
#5058=DIRECTION('ref_axis',(1.,0.,0.));
#5059=DIRECTION('center_axis',(0.,1.,0.));
#5060=DIRECTION('ref_axis',(-1.,0.,0.));
#5061=DIRECTION('',(-1.,0.,0.));
#5062=DIRECTION('',(0.,0.,1.));
#5063=DIRECTION('',(0.,0.,1.));
#5064=DIRECTION('center_axis',(0.,0.,-1.));
#5065=DIRECTION('ref_axis',(0.,1.,0.));
#5066=DIRECTION('center_axis',(0.,0.,1.));
#5067=DIRECTION('ref_axis',(0.,1.,0.));
#5068=DIRECTION('',(0.,0.,1.));
#5069=DIRECTION('center_axis',(0.,-1.,0.));
#5070=DIRECTION('ref_axis',(1.,0.,0.));
#5071=DIRECTION('',(1.,0.,0.));
#5072=DIRECTION('',(0.,0.,1.));
#5073=DIRECTION('center_axis',(0.,0.,-1.));
#5074=DIRECTION('ref_axis',(0.,-1.,0.));
#5075=DIRECTION('center_axis',(0.,0.,1.));
#5076=DIRECTION('ref_axis',(0.,-1.,0.));
#5077=DIRECTION('center_axis',(0.,1.,0.));
#5078=DIRECTION('ref_axis',(-1.,0.,0.));
#5079=DIRECTION('',(-1.,0.,0.));
#5080=DIRECTION('',(0.,0.,1.));
#5081=DIRECTION('',(0.,0.,1.));
#5082=DIRECTION('center_axis',(0.,0.,-1.));
#5083=DIRECTION('ref_axis',(0.,1.,0.));
#5084=DIRECTION('center_axis',(0.,0.,1.));
#5085=DIRECTION('ref_axis',(0.,1.,0.));
#5086=DIRECTION('',(0.,0.,1.));
#5087=DIRECTION('center_axis',(0.,-1.,0.));
#5088=DIRECTION('ref_axis',(1.,0.,0.));
#5089=DIRECTION('',(1.,0.,0.));
#5090=DIRECTION('',(0.,0.,1.));
#5091=DIRECTION('center_axis',(0.,0.,-1.));
#5092=DIRECTION('ref_axis',(0.,-1.,0.));
#5093=DIRECTION('center_axis',(0.,0.,1.));
#5094=DIRECTION('ref_axis',(0.,-1.,0.));
#5095=DIRECTION('center_axis',(1.,-3.51417407375166E-16,0.));
#5096=DIRECTION('ref_axis',(3.51417407375166E-16,1.,0.));
#5097=DIRECTION('',(0.,0.,1.));
#5098=DIRECTION('',(0.,1.,0.));
#5099=DIRECTION('center_axis',(0.,0.,-1.));
#5100=DIRECTION('ref_axis',(3.55271367880049E-15,1.,0.));
#5101=DIRECTION('center_axis',(0.,0.,-1.));
#5102=DIRECTION('ref_axis',(3.55271367880049E-15,1.,0.));
#5103=DIRECTION('',(0.,0.,1.));
#5104=DIRECTION('center_axis',(2.36032074788338E-16,-1.,0.));
#5105=DIRECTION('ref_axis',(1.,2.36032074788338E-16,0.));
#5106=DIRECTION('',(-1.,-2.36032074788338E-16,0.));
#5107=DIRECTION('',(0.,0.,1.));
#5108=DIRECTION('center_axis',(0.,0.,-1.));
#5109=DIRECTION('ref_axis',(-1.,0.,0.));
#5110=DIRECTION('center_axis',(0.,0.,-1.));
#5111=DIRECTION('ref_axis',(-1.,0.,0.));
#5112=DIRECTION('center_axis',(0.,0.,-1.));
#5113=DIRECTION('ref_axis',(1.,0.,0.));
#6002=CARTESIAN_POINT('',(0.,0.,0.));
#6003=CARTESIAN_POINT('Origin',(24.7143466872546,3.13165946910082,-0.395297377936459));
#6004=CARTESIAN_POINT('',(24.7143466872546,3.63165946910083,1.30603779103116));
#6005=CARTESIAN_POINT('Origin',(24.7143466872546,3.63165946910082,-0.395297377936459));
#6006=CARTESIAN_POINT('',(24.7143466872546,3.13165946910082,1.80603779103116));
#6007=CARTESIAN_POINT('Origin',(24.7143466872546,3.13165946910082,1.30603779103116));
#6008=CARTESIAN_POINT('Origin',(24.7143466872546,3.13165946910082,-0.395297377936459));
#6009=CARTESIAN_POINT('Origin',(24.7143466872546,3.63165946910082,-0.395297377936459));
#6010=CARTESIAN_POINT('Origin',(37.3390884548007,3.13165946910082,-0.451167579126729));
#6011=CARTESIAN_POINT('',(37.3390884548007,3.63165946910083,1.30858121201868));
#6012=CARTESIAN_POINT('Origin',(37.3390884548007,3.63165946910082,-0.451167579126729));
#6013=CARTESIAN_POINT('',(37.3390884548007,3.13165946910082,1.80858121201868));
#6014=CARTESIAN_POINT('Origin',(37.3390884548007,3.13165946910082,1.30858121201868));
#6015=CARTESIAN_POINT('Origin',(37.3390884548007,3.13165946910082,-0.451167579126729));
#6016=CARTESIAN_POINT('Origin',(37.3390884548007,3.63165946910082,-0.451167579126729));
#6017=CARTESIAN_POINT('Origin',(25.1607982446856,4.63165946910082,-5.));
#6018=CARTESIAN_POINT('',(19.2071026744088,4.63165946910082,-6.5));
#6019=CARTESIAN_POINT('',(19.8239560216472,3.13165946910082,-5.));
#6020=CARTESIAN_POINT('Origin',(19.8239560216472,4.63165946910082,-5.));
#6021=CARTESIAN_POINT('',(42.4050316082777,3.13165946910082,-5.));
#6022=CARTESIAN_POINT('',(25.1607982446856,3.13165946910082,-5.));
#6023=CARTESIAN_POINT('',(43.0218849555161,4.63165946910082,-6.5));
#6024=CARTESIAN_POINT('Origin',(42.4050316082777,4.63165946910082,-5.));
#6025=CARTESIAN_POINT('',(25.1607982446856,4.63165946910082,-6.5));
#6026=CARTESIAN_POINT('Origin',(31.1144938149625,7.54093103995931,-6.5));
#6027=CARTESIAN_POINT('',(43.0218849555161,9.4502026108178,-6.5));
#6028=CARTESIAN_POINT('',(43.0218849555161,3.13165946910082,-6.5));
#6029=CARTESIAN_POINT('',(40.5218849555161,11.9502026108178,-6.5));
#6030=CARTESIAN_POINT('Origin',(40.5218849555161,9.45020261081779,-6.5));
#6031=CARTESIAN_POINT('',(21.7071026744088,11.9502026108178,-6.5));
#6032=CARTESIAN_POINT('',(40.5218849555161,11.9502026108178,-6.5));
#6033=CARTESIAN_POINT('',(19.2071026744088,9.4502026108178,-6.5));
#6034=CARTESIAN_POINT('Origin',(21.7071026744088,9.4502026108178,-6.5));
#6035=CARTESIAN_POINT('',(19.2071026744088,9.4502026108178,-6.5));
#6036=CARTESIAN_POINT('',(36.8121029357457,10.3406188648021,-6.5));
#6037=CARTESIAN_POINT('',(36.8121029357457,5.74734553320186,-6.5));
#6038=CARTESIAN_POINT('Origin',(36.8121029357457,8.04398219900198,-6.5));
#6039=CARTESIAN_POINT('',(38.9466240721952,10.3406188648021,-6.5));
#6040=CARTESIAN_POINT('',(36.8121029357457,10.3406188648021,-6.5));
#6041=CARTESIAN_POINT('',(38.9466240721952,5.74734553320186,-6.5));
#6042=CARTESIAN_POINT('Origin',(38.9466240721952,8.04398219900198,-6.5));
#6043=CARTESIAN_POINT('',(38.9466240721952,5.74734553320186,-6.5));
#6044=CARTESIAN_POINT('',(23.3121029357457,10.3406188648021,-6.5));
#6045=CARTESIAN_POINT('',(23.3121029357457,5.74734553320186,-6.5));
#6046=CARTESIAN_POINT('Origin',(23.3121029357457,8.04398219900198,-6.5));
#6047=CARTESIAN_POINT('',(25.4466240721952,10.3406188648021,-6.5));
#6048=CARTESIAN_POINT('',(23.3121029357457,10.3406188648021,-6.5));
#6049=CARTESIAN_POINT('',(25.4466240721952,5.74734553320186,-6.5));
#6050=CARTESIAN_POINT('Origin',(25.4466240721952,8.04398219900198,-6.5));
#6051=CARTESIAN_POINT('',(25.4466240721952,5.74734553320186,-6.5));
#6052=CARTESIAN_POINT('Origin',(37.2590007645168,2.75665946910082,0.));
#6053=CARTESIAN_POINT('',(34.7590007645168,3.13165946910082,0.));
#6054=CARTESIAN_POINT('',(37.2590007645168,3.13165946910082,2.5));
#6055=CARTESIAN_POINT('Origin',(37.2590007645168,3.13165946910082,0.));
#6056=CARTESIAN_POINT('',(34.7590007645168,1.63165946910082,0.));
#6057=CARTESIAN_POINT('',(34.7590007645168,2.75665946910082,0.));
#6058=CARTESIAN_POINT('',(37.2590007645168,1.63165946910082,2.5));
#6059=CARTESIAN_POINT('Origin',(37.2590007645168,1.63165946910082,0.));
#6060=CARTESIAN_POINT('',(37.2590007645168,2.75665946910082,2.5));
#6061=CARTESIAN_POINT('Origin',(31.1144938149625,2.38165946910082,2.5));
#6062=CARTESIAN_POINT('',(37.4782084817555,1.63165946910082,2.5));
#6063=CARTESIAN_POINT('',(43.0218849555161,1.63165946910082,2.5));
#6064=CARTESIAN_POINT('',(37.4782084817555,3.13165946910082,2.5));
#6065=CARTESIAN_POINT('',(37.4782084817555,2.75665946910082,2.5));
#6066=CARTESIAN_POINT('',(19.2071026744088,3.13165946910082,2.5));
#6067=CARTESIAN_POINT('Origin',(19.2071026744088,3.13165946910082,-8.5));
#6068=CARTESIAN_POINT('',(22.2074408259328,3.13165946910082,0.795911171487552));
#6069=CARTESIAN_POINT('',(20.7059131671521,3.13165946910082,-2.85534807555141));
#6070=CARTESIAN_POINT('',(24.7507791481694,3.13165946910082,2.5));
#6071=CARTESIAN_POINT('Origin',(24.7507791481694,3.13165946910082,-0.25));
#6072=CARTESIAN_POINT('',(24.9699868654081,3.13165946910082,2.5));
#6073=CARTESIAN_POINT('',(19.2071026744088,3.13165946910082,2.5));
#6074=CARTESIAN_POINT('',(27.4699868654081,3.13165946910082,0.));
#6075=CARTESIAN_POINT('Origin',(24.9699868654081,3.13165946910082,0.));
#6076=CARTESIAN_POINT('',(27.4699868654081,3.13165946910082,-0.758936728277321));
#6077=CARTESIAN_POINT('',(27.4699868654081,3.13165946910082,-4.62946836413866));
#6078=CARTESIAN_POINT('',(27.5384895461752,3.13165946910082,-1.277895402736));
#6079=CARTESIAN_POINT('Origin',(29.4699868654084,3.13165946910082,-0.758936728277284));
#6080=CARTESIAN_POINT('',(34.6904980837498,3.13165946910082,-1.277895402736));
#6081=CARTESIAN_POINT('Origin',(31.1144938149625,3.13165946910082,-0.317087216926334));
#6082=CARTESIAN_POINT('',(34.7590007645168,3.13165946910082,-0.758936728277321));
#6083=CARTESIAN_POINT('Origin',(32.7590007645165,3.13165946910082,-0.758936728277284));
#6084=CARTESIAN_POINT('',(34.7590007645168,3.13165946910082,-3.));
#6085=CARTESIAN_POINT('',(40.0215468039921,3.13165946910082,0.79591117148755));
#6086=CARTESIAN_POINT('Origin',(37.4782084817555,3.13165946910082,-0.25));
#6087=CARTESIAN_POINT('',(41.6512074608448,3.13165946910082,-3.16692861243009));
#6088=CARTESIAN_POINT('Origin',(24.9699868654081,2.75665946910082,0.));
#6089=CARTESIAN_POINT('',(27.4699868654081,1.63165946910082,0.));
#6090=CARTESIAN_POINT('',(24.9699868654081,1.63165946910082,2.5));
#6091=CARTESIAN_POINT('Origin',(24.9699868654081,1.63165946910082,0.));
#6092=CARTESIAN_POINT('',(27.4699868654081,2.75665946910082,0.));
#6093=CARTESIAN_POINT('',(24.9699868654081,2.75665946910082,2.5));
#6094=CARTESIAN_POINT('Origin',(27.4699868654081,3.13165946910082,-0.758936728277321));
#6095=CARTESIAN_POINT('',(27.4699868654081,1.63165946910082,-0.758936728277321));
#6096=CARTESIAN_POINT('',(27.4699868654081,1.63165946910082,-4.62946836413866));
#6097=CARTESIAN_POINT('',(27.4699868654081,3.13165946910082,-0.758936728277321));
#6098=CARTESIAN_POINT('Origin',(37.4782084817555,2.75665946910082,-0.25));
#6099=CARTESIAN_POINT('',(40.0215468039921,1.63165946910082,0.795911171487551));
#6100=CARTESIAN_POINT('Origin',(37.4782084817555,1.63165946910082,-0.25));
#6101=CARTESIAN_POINT('',(40.0215468039921,2.75665946910082,0.795911171487553));
#6102=CARTESIAN_POINT('Origin',(43.0218849555161,3.13165946910082,-6.5));
#6103=CARTESIAN_POINT('',(43.0218849555161,1.63165946910082,-6.5));
#6104=CARTESIAN_POINT('',(43.373634504488,1.63165946910082,-7.35534807555141));
#6105=CARTESIAN_POINT('',(43.0218849555161,3.13165946910082,-6.5));
#6106=CARTESIAN_POINT('Origin',(24.7507791481694,2.75665946910082,-0.25));
#6107=CARTESIAN_POINT('',(22.2074408259328,1.63165946910082,0.795911171487552));
#6108=CARTESIAN_POINT('',(22.2074408259328,2.75665946910082,0.795911171487551));
#6109=CARTESIAN_POINT('',(24.7507791481694,1.63165946910082,2.5));
#6110=CARTESIAN_POINT('Origin',(24.7507791481694,1.63165946910082,-0.25));
#6111=CARTESIAN_POINT('',(24.7507791481694,2.75665946910082,2.5));
#6112=CARTESIAN_POINT('Origin',(22.9082227578391,3.13165946910082,2.5));
#6113=CARTESIAN_POINT('',(19.2071026744088,1.63165946910082,-6.5));
#6114=CARTESIAN_POINT('',(19.2071026744088,3.13165946910083,-6.5));
#6115=CARTESIAN_POINT('',(22.4283402107953,1.63165946910082,1.3330713875699));
#6116=CARTESIAN_POINT('Origin',(32.7590007645165,3.13165946910082,-0.758936728277284));
#6117=CARTESIAN_POINT('',(34.6904980837498,1.63165946910082,-1.277895402736));
#6118=CARTESIAN_POINT('',(34.7590007645168,1.63165946910082,-0.758936728277321));
#6119=CARTESIAN_POINT('Origin',(32.7590007645165,1.63165946910082,-0.758936728277284));
#6120=CARTESIAN_POINT('',(34.7590007645168,3.13165946910082,-0.758936728277321));
#6121=CARTESIAN_POINT('',(34.6904980837498,3.13165946910082,-1.277895402736));
#6122=CARTESIAN_POINT('Origin',(34.7590007645168,3.13165946910082,2.5));
#6123=CARTESIAN_POINT('',(34.7590007645168,1.63165946910082,-3.));
#6124=CARTESIAN_POINT('Origin',(29.4699868654084,3.13165946910082,-0.758936728277284));
#6125=CARTESIAN_POINT('',(27.5384895461752,1.63165946910082,-1.277895402736));
#6126=CARTESIAN_POINT('Origin',(29.4699868654084,1.63165946910082,-0.758936728277284));
#6127=CARTESIAN_POINT('',(27.5384895461752,3.13165946910082,-1.277895402736));
#6128=CARTESIAN_POINT('Origin',(31.1144938149625,3.13165946910082,-0.317087216926334));
#6129=CARTESIAN_POINT('Origin',(31.1144938149625,1.63165946910082,-0.317087216926334));
#6130=CARTESIAN_POINT('Origin',(43.0218849555161,9.4502026108178,-8.5));
#6131=CARTESIAN_POINT('',(43.0218849555161,1.63165946910082,-8.5));
#6132=CARTESIAN_POINT('',(43.0218849555161,1.63165946910082,-8.5));
#6133=CARTESIAN_POINT('',(43.0218849555161,9.4502026108178,-8.5));
#6134=CARTESIAN_POINT('',(43.0218849555161,3.13165946910082,-8.5));
#6135=CARTESIAN_POINT('',(43.0218849555161,9.4502026108178,-8.5));
#6136=CARTESIAN_POINT('Origin',(43.0218849555161,1.63165946910082,-8.5));
#6137=CARTESIAN_POINT('',(43.0218849555161,1.63165946910082,2.5));
#6138=CARTESIAN_POINT('',(19.2071026744088,1.63165946910082,-8.5));
#6139=CARTESIAN_POINT('',(19.2071026744088,1.63165946910082,-8.5));
#6140=CARTESIAN_POINT('',(43.0218849555161,1.63165946910082,-8.5));
#6141=CARTESIAN_POINT('Origin',(31.1144938149625,2.38165946910082,2.5));
#6142=CARTESIAN_POINT('Origin',(38.9466240721952,10.3406188648021,-8.5));
#6143=CARTESIAN_POINT('',(38.9466240721952,10.3406188648021,-8.5));
#6144=CARTESIAN_POINT('',(36.8121029357457,10.3406188648021,-8.5));
#6145=CARTESIAN_POINT('',(36.8121029357457,10.3406188648021,-8.5));
#6146=CARTESIAN_POINT('',(38.9466240721952,10.3406188648021,-8.5));
#6147=CARTESIAN_POINT('',(36.8121029357457,10.3406188648021,-8.5));
#6148=CARTESIAN_POINT('Origin',(38.9466240721952,8.04398219900198,-8.5));
#6149=CARTESIAN_POINT('',(38.9466240721952,5.74734553320186,-8.5));
#6150=CARTESIAN_POINT('Origin',(38.9466240721952,8.04398219900198,-8.5));
#6151=CARTESIAN_POINT('',(38.9466240721952,5.74734553320186,-8.5));
#6152=CARTESIAN_POINT('Origin',(36.8121029357457,5.74734553320186,-8.5));
#6153=CARTESIAN_POINT('',(36.8121029357457,5.74734553320186,-8.5));
#6154=CARTESIAN_POINT('',(38.9466240721952,5.74734553320186,-8.5));
#6155=CARTESIAN_POINT('',(36.8121029357457,5.74734553320186,-8.5));
#6156=CARTESIAN_POINT('Origin',(36.8121029357457,8.04398219900198,-8.5));
#6157=CARTESIAN_POINT('Origin',(36.8121029357457,8.04398219900198,-8.5));
#6158=CARTESIAN_POINT('Origin',(25.4466240721952,10.3406188648021,-8.5));
#6159=CARTESIAN_POINT('',(25.4466240721952,10.3406188648021,-8.5));
#6160=CARTESIAN_POINT('',(23.3121029357457,10.3406188648021,-8.5));
#6161=CARTESIAN_POINT('',(23.3121029357457,10.3406188648021,-8.5));
#6162=CARTESIAN_POINT('',(25.4466240721952,10.3406188648021,-8.5));
#6163=CARTESIAN_POINT('',(23.3121029357457,10.3406188648021,-8.5));
#6164=CARTESIAN_POINT('Origin',(25.4466240721952,8.04398219900198,-8.5));
#6165=CARTESIAN_POINT('',(25.4466240721952,5.74734553320186,-8.5));
#6166=CARTESIAN_POINT('Origin',(25.4466240721952,8.04398219900198,-8.5));
#6167=CARTESIAN_POINT('',(25.4466240721952,5.74734553320186,-8.5));
#6168=CARTESIAN_POINT('Origin',(23.3121029357457,5.74734553320186,-8.5));
#6169=CARTESIAN_POINT('',(23.3121029357457,5.74734553320186,-8.5));
#6170=CARTESIAN_POINT('',(25.4466240721952,5.74734553320186,-8.5));
#6171=CARTESIAN_POINT('',(23.3121029357457,5.74734553320186,-8.5));
#6172=CARTESIAN_POINT('Origin',(23.3121029357457,8.04398219900198,-8.5));
#6173=CARTESIAN_POINT('Origin',(23.3121029357457,8.04398219900198,-8.5));
#6174=CARTESIAN_POINT('Origin',(19.2071026744088,3.13165946910082,-8.5));
#6175=CARTESIAN_POINT('',(19.2071026744088,9.4502026108178,-8.5));
#6176=CARTESIAN_POINT('',(19.2071026744088,9.4502026108178,-8.5));
#6177=CARTESIAN_POINT('',(19.2071026744088,1.63165946910082,-8.5));
#6178=CARTESIAN_POINT('Origin',(40.5218849555161,9.45020261081779,-8.5));
#6179=CARTESIAN_POINT('',(40.5218849555161,11.9502026108178,-8.5));
#6180=CARTESIAN_POINT('Origin',(40.5218849555161,9.45020261081779,-8.5));
#6181=CARTESIAN_POINT('',(40.5218849555161,11.9502026108178,-8.5));
#6182=CARTESIAN_POINT('Origin',(21.7071026744088,11.9502026108178,-8.5));
#6183=CARTESIAN_POINT('',(21.7071026744088,11.9502026108178,-8.5));
#6184=CARTESIAN_POINT('',(40.5218849555161,11.9502026108178,-8.5));
#6185=CARTESIAN_POINT('',(21.7071026744088,11.9502026108178,-8.5));
#6186=CARTESIAN_POINT('Origin',(21.7071026744088,9.4502026108178,-8.5));
#6187=CARTESIAN_POINT('Origin',(21.7071026744088,9.4502026108178,-8.5));
#6188=CARTESIAN_POINT('Origin',(31.1144938149625,7.54093103995931,-8.5));
#23559=UNCERTAINTY_MEASURE_WITH_UNIT(LENGTH_MEASURE(0.01),#23578,
'DISTANCE_ACCURACY_VALUE',
'Maximum model space distance between geometric entities at asserted c
onnectivities');
#23566=UNCERTAINTY_MEASURE_WITH_UNIT(LENGTH_MEASURE(0.01),#23578,
'DISTANCE_ACCURACY_VALUE',
'Maximum model space distance between geometric entities at asserted c
onnectivities');
#23570=(
GEOMETRIC_REPRESENTATION_CONTEXT(3)
GLOBAL_UNCERTAINTY_ASSIGNED_CONTEXT((#23559))
GLOBAL_UNIT_ASSIGNED_CONTEXT((#23578,#23580,#23581))
REPRESENTATION_CONTEXT('','3D')
);
#23577=(
GEOMETRIC_REPRESENTATION_CONTEXT(3)
GLOBAL_UNCERTAINTY_ASSIGNED_CONTEXT((#23566))
GLOBAL_UNIT_ASSIGNED_CONTEXT((#23578,#23580,#23581))
REPRESENTATION_CONTEXT('','3D')
);
#23578=(
LENGTH_UNIT()
NAMED_UNIT(*)
SI_UNIT(.MILLI.,.METRE.)
);
#23580=(
NAMED_UNIT(*)
PLANE_ANGLE_UNIT()
SI_UNIT($,.RADIAN.)
);
#23581=(
NAMED_UNIT(*)
SI_UNIT($,.STERADIAN.)
SOLID_ANGLE_UNIT()
);
#23585=SHAPE_DEFINITION_REPRESENTATION(#23595,#23614);
#23595=PRODUCT_DEFINITION_SHAPE('',$,#23625);
#23614=SHAPE_REPRESENTATION('',(#4354),#23570);
#23621=PRODUCT_DEFINITION_CONTEXT('part definition',#23653,'design');
#23625=PRODUCT_DEFINITION('Base_Right','Base_Right',#23635,#23621);
#23635=PRODUCT_DEFINITION_FORMATION('',$,#23658);
#23653=APPLICATION_CONTEXT(
'Core Data for Automotive Mechanical Design Process');
#23654=PRODUCT_CONTEXT('part definition',#23653,'mechanical');
#23658=PRODUCT('Base_Right','Base_Right',$,(#23654));
#23666=PRESENTATION_STYLE_ASSIGNMENT((#23671));
#23671=SURFACE_STYLE_USAGE(.BOTH.,#23676);
#23676=SURFACE_SIDE_STYLE('',(#23681));
#23681=SURFACE_STYLE_FILL_AREA(#23686);
#23686=FILL_AREA_STYLE('Opaque(210,210,210)',(#23691));
#23691=FILL_AREA_STYLE_COLOUR('Opaque(210,210,210)',#23696);
#23696=COLOUR_RGB('Opaque(210,210,210)', 0.09019608, 0.27058824, 0.51372549);
ENDSEC;
END-ISO-10303-21;
